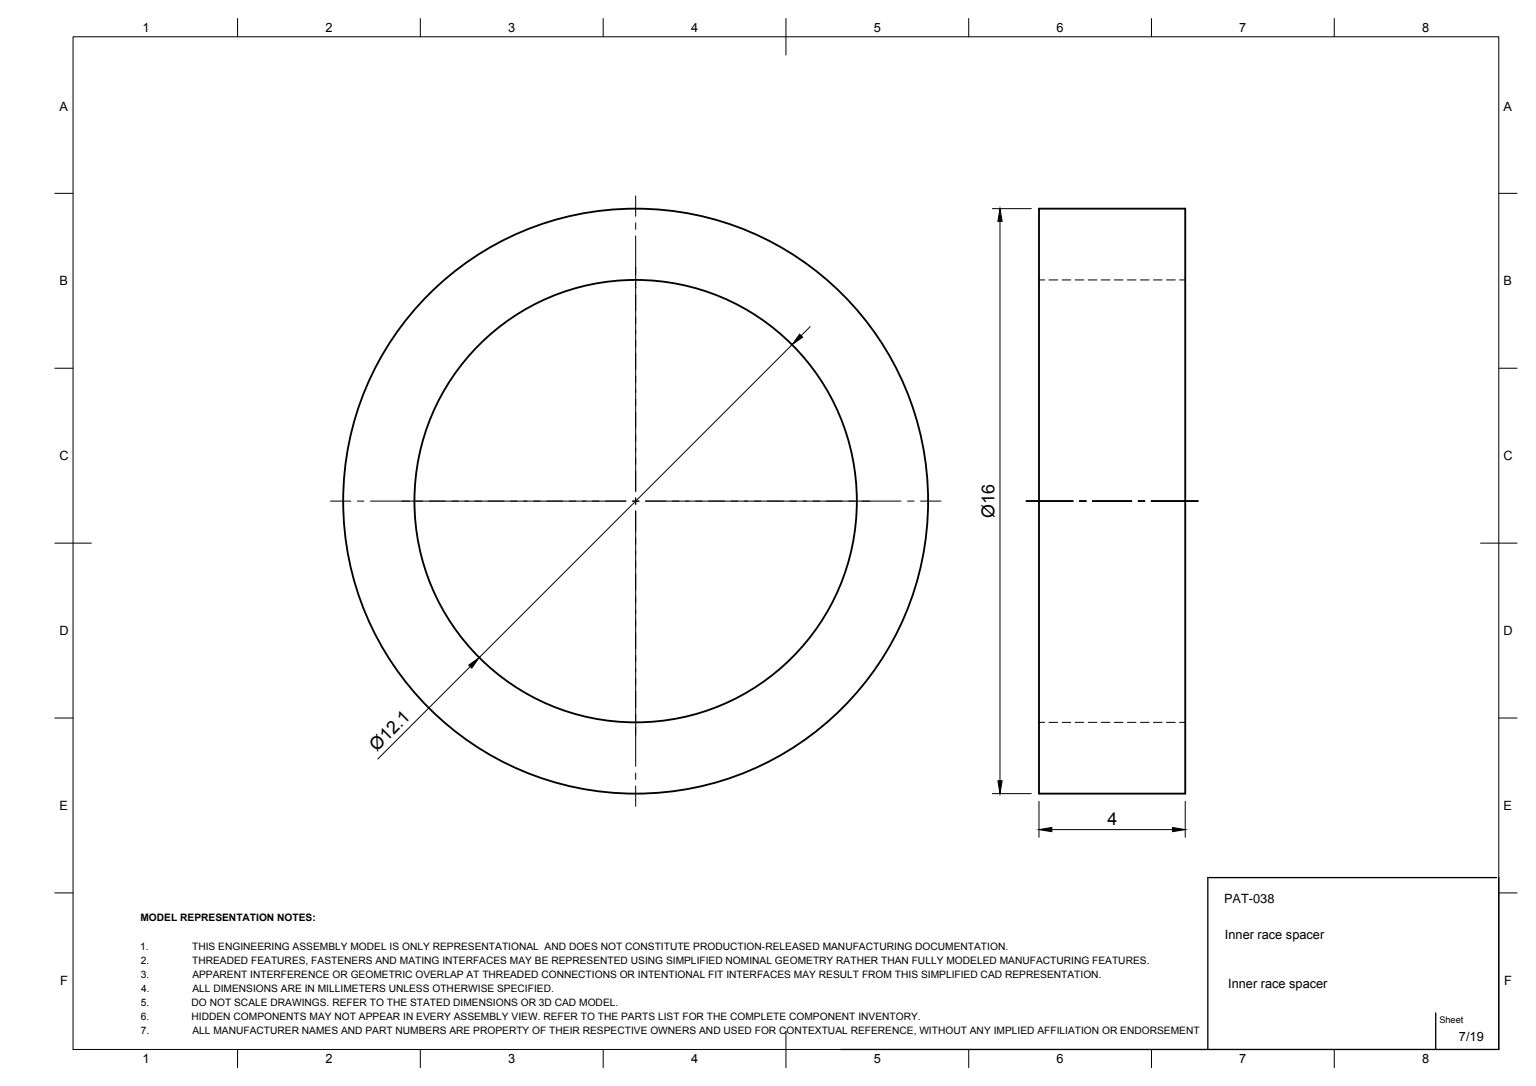
ISO-10303-21;
HEADER;
/* Generated by software containing ST-Developer
 * from STEP Tools, Inc. (www.steptools.com) 
 */

FILE_DESCRIPTION(
/* description */ ('Fork-mounted skate wheel'),
/* implementation_level */ '2;1');

FILE_NAME(
/* name */ 'Inner race spacer.step',
/* time_stamp */ '2026-10-29T16:11:26-07:00',
/* author */ (''),
/* organization */ (''),
/* preprocessor_version */ 'ST-DEVELOPER v20.2',
/* originating_system */ 'Autodesk Translation Framework v15.17.0.0',
/* authorisation */ '');

FILE_SCHEMA (('AUTOMOTIVE_DESIGN { 1 0 10303 214 3 1 1 }'));
ENDSEC;

DATA;
#10=MECHANICAL_DESIGN_GEOMETRIC_PRESENTATION_REPRESENTATION('',(#148),#3688);
#124=SHAPE_REPRESENTATION_RELATIONSHIP('SRR','None',#3747,#136);
#136=ADVANCED_BREP_SHAPE_REPRESENTATION('',(#167),#3676);
#148=STYLED_ITEM('',(#3896),#167);
#167=MANIFOLD_SOLID_BREP('Body1',#1809);
#199=FACE_BOUND('',#437,.T.);
#200=FACE_BOUND('',#439,.T.);
#239=PLANE('',#2018);
#240=PLANE('',#2019);
#305=FACE_OUTER_BOUND('',#434,.T.);
#306=FACE_OUTER_BOUND('',#435,.T.);
#307=FACE_OUTER_BOUND('',#436,.T.);
#308=FACE_OUTER_BOUND('',#438,.T.);
#434=EDGE_LOOP('',(#1343,#1344,#1345,#1346));
#435=EDGE_LOOP('',(#1347,#1348,#1349,#1350));
#436=EDGE_LOOP('',(#1351));
#437=EDGE_LOOP('',(#1352));
#438=EDGE_LOOP('',(#1353));
#439=EDGE_LOOP('',(#1354));
#583=LINE('',#2980,#677);
#584=LINE('',#2986,#678);
#677=VECTOR('',#2374,0.605);
#678=VECTOR('',#2381,0.8);
#744=CIRCLE('',#2013,0.605);
#745=CIRCLE('',#2014,0.605);
#746=CIRCLE('',#2016,0.8);
#747=CIRCLE('',#2017,0.8);
#882=VERTEX_POINT('',#2977);
#883=VERTEX_POINT('',#2979);
#884=VERTEX_POINT('',#2983);
#885=VERTEX_POINT('',#2985);
#1058=EDGE_CURVE('',#882,#882,#744,.T.);
#1059=EDGE_CURVE('',#882,#883,#583,.T.);
#1060=EDGE_CURVE('',#883,#883,#745,.T.);
#1061=EDGE_CURVE('',#884,#884,#746,.T.);
#1062=EDGE_CURVE('',#884,#885,#584,.T.);
#1063=EDGE_CURVE('',#885,#885,#747,.T.);
#1343=ORIENTED_EDGE('',*,*,#1058,.F.);
#1344=ORIENTED_EDGE('',*,*,#1059,.T.);
#1345=ORIENTED_EDGE('',*,*,#1060,.T.);
#1346=ORIENTED_EDGE('',*,*,#1059,.F.);
#1347=ORIENTED_EDGE('',*,*,#1061,.F.);
#1348=ORIENTED_EDGE('',*,*,#1062,.T.);
#1349=ORIENTED_EDGE('',*,*,#1063,.T.);
#1350=ORIENTED_EDGE('',*,*,#1062,.F.);
#1351=ORIENTED_EDGE('',*,*,#1061,.T.);
#1352=ORIENTED_EDGE('',*,*,#1058,.T.);
#1353=ORIENTED_EDGE('',*,*,#1063,.F.);
#1354=ORIENTED_EDGE('',*,*,#1060,.F.);
#1670=CYLINDRICAL_SURFACE('',#2012,0.605);
#1671=CYLINDRICAL_SURFACE('',#2015,0.8);
#1723=ADVANCED_FACE('',(#305),#1670,.F.);
#1724=ADVANCED_FACE('',(#306),#1671,.T.);
#1725=ADVANCED_FACE('',(#307,#199),#239,.T.);
#1726=ADVANCED_FACE('',(#308,#200),#240,.F.);
#1809=CLOSED_SHELL('',(#1723,#1724,#1725,#1726));
#2011=AXIS2_PLACEMENT_3D('',#2975,#2368,#2369);
#2012=AXIS2_PLACEMENT_3D('',#2976,#2370,#2371);
#2013=AXIS2_PLACEMENT_3D('',#2978,#2372,#2373);
#2014=AXIS2_PLACEMENT_3D('',#2981,#2375,#2376);
#2015=AXIS2_PLACEMENT_3D('',#2982,#2377,#2378);
#2016=AXIS2_PLACEMENT_3D('',#2984,#2379,#2380);
#2017=AXIS2_PLACEMENT_3D('',#2987,#2382,#2383);
#2018=AXIS2_PLACEMENT_3D('',#2988,#2384,#2385);
#2019=AXIS2_PLACEMENT_3D('',#2989,#2386,#2387);
#2368=DIRECTION('axis',(0.,0.,1.));
#2369=DIRECTION('refdir',(1.,0.,0.));
#2370=DIRECTION('center_axis',(0.,1.,0.));
#2371=DIRECTION('ref_axis',(1.,0.,0.));
#2372=DIRECTION('center_axis',(0.,-1.,0.));
#2373=DIRECTION('ref_axis',(1.,0.,0.));
#2374=DIRECTION('',(0.,-1.,0.));
#2375=DIRECTION('center_axis',(0.,-1.,0.));
#2376=DIRECTION('ref_axis',(1.,0.,0.));
#2377=DIRECTION('center_axis',(0.,1.,0.));
#2378=DIRECTION('ref_axis',(1.,0.,0.));
#2379=DIRECTION('center_axis',(0.,1.,0.));
#2380=DIRECTION('ref_axis',(1.,0.,0.));
#2381=DIRECTION('',(0.,-1.,0.));
#2382=DIRECTION('center_axis',(0.,1.,0.));
#2383=DIRECTION('ref_axis',(1.,0.,0.));
#2384=DIRECTION('center_axis',(0.,1.,0.));
#2385=DIRECTION('ref_axis',(1.,0.,0.));
#2386=DIRECTION('center_axis',(0.,1.,0.));
#2387=DIRECTION('ref_axis',(1.,0.,0.));
#2975=CARTESIAN_POINT('',(0.,0.,0.));
#2976=CARTESIAN_POINT('Origin',(0.,4.5,10.));
#2977=CARTESIAN_POINT('',(-0.605,4.9,10.));
#2978=CARTESIAN_POINT('Origin',(0.,4.9,10.));
#2979=CARTESIAN_POINT('',(-0.605,4.5,10.));
#2980=CARTESIAN_POINT('',(-0.605,4.5,10.));
#2981=CARTESIAN_POINT('Origin',(0.,4.5,10.));
#2982=CARTESIAN_POINT('Origin',(0.,4.5,10.));
#2983=CARTESIAN_POINT('',(-0.8,4.9,10.));
#2984=CARTESIAN_POINT('Origin',(0.,4.9,10.));
#2985=CARTESIAN_POINT('',(-0.8,4.5,10.));
#2986=CARTESIAN_POINT('',(-0.8,4.5,10.));
#2987=CARTESIAN_POINT('Origin',(0.,4.5,10.));
#2988=CARTESIAN_POINT('Origin',(0.,4.9,10.));
#2989=CARTESIAN_POINT('Origin',(0.,4.5,10.));
#3659=UNCERTAINTY_MEASURE_WITH_UNIT(LENGTH_MEASURE(0.001),#3689,
'DISTANCE_ACCURACY_VALUE',
'Maximum model space distance between geometric entities at asserted c
onnectivities');
#3671=UNCERTAINTY_MEASURE_WITH_UNIT(LENGTH_MEASURE(0.001),#3689,
'DISTANCE_ACCURACY_VALUE',
'Maximum model space distance between geometric entities at asserted c
onnectivities');
#3676=(
GEOMETRIC_REPRESENTATION_CONTEXT(3)
GLOBAL_UNCERTAINTY_ASSIGNED_CONTEXT((#3659))
GLOBAL_UNIT_ASSIGNED_CONTEXT((#3689,#3691,#3692))
REPRESENTATION_CONTEXT('','3D')
);
#3688=(
GEOMETRIC_REPRESENTATION_CONTEXT(3)
GLOBAL_UNCERTAINTY_ASSIGNED_CONTEXT((#3671))
GLOBAL_UNIT_ASSIGNED_CONTEXT((#3689,#3691,#3692))
REPRESENTATION_CONTEXT('','3D')
);
#3689=(
LENGTH_UNIT()
NAMED_UNIT(*)
SI_UNIT(.CENTI.,.METRE.)
);
#3691=(
NAMED_UNIT(*)
PLANE_ANGLE_UNIT()
SI_UNIT($,.RADIAN.)
);
#3692=(
NAMED_UNIT(*)
SI_UNIT($,.STERADIAN.)
SOLID_ANGLE_UNIT()
);
#3697=SHAPE_DEFINITION_REPRESENTATION(#3713,#3747);
#3713=PRODUCT_DEFINITION_SHAPE('',$,#3764);
#3747=SHAPE_REPRESENTATION('',(#2011),#3676);
#3759=PRODUCT_DEFINITION_CONTEXT('part definition',#3809,'design');
#3764=PRODUCT_DEFINITION('Inner race spacer','Inner race spacer',#3780,
#3759);
#3780=PRODUCT_DEFINITION_FORMATION('',$,#3815);
#3809=APPLICATION_CONTEXT(
'Core Data for Automotive Mechanical Design Process');
#3810=PRODUCT_CONTEXT('part definition',#3809,'mechanical');
#3815=PRODUCT('Inner race spacer','Inner race spacer',
'Inner race spacer',(#3810));
#3890=COLOUR_RGB('Grey',0.48,0.52,0.57);
#3891=FILL_AREA_STYLE_COLOUR('',#3890);
#3892=FILL_AREA_STYLE('',(#3891));
#3893=SURFACE_STYLE_FILL_AREA(#3892);
#3894=SURFACE_SIDE_STYLE('',(#3893));
#3895=SURFACE_STYLE_USAGE(.BOTH.,#3894);
#3896=PRESENTATION_STYLE_ASSIGNMENT((#3895));
ENDSEC;
END-ISO-10303-21;
